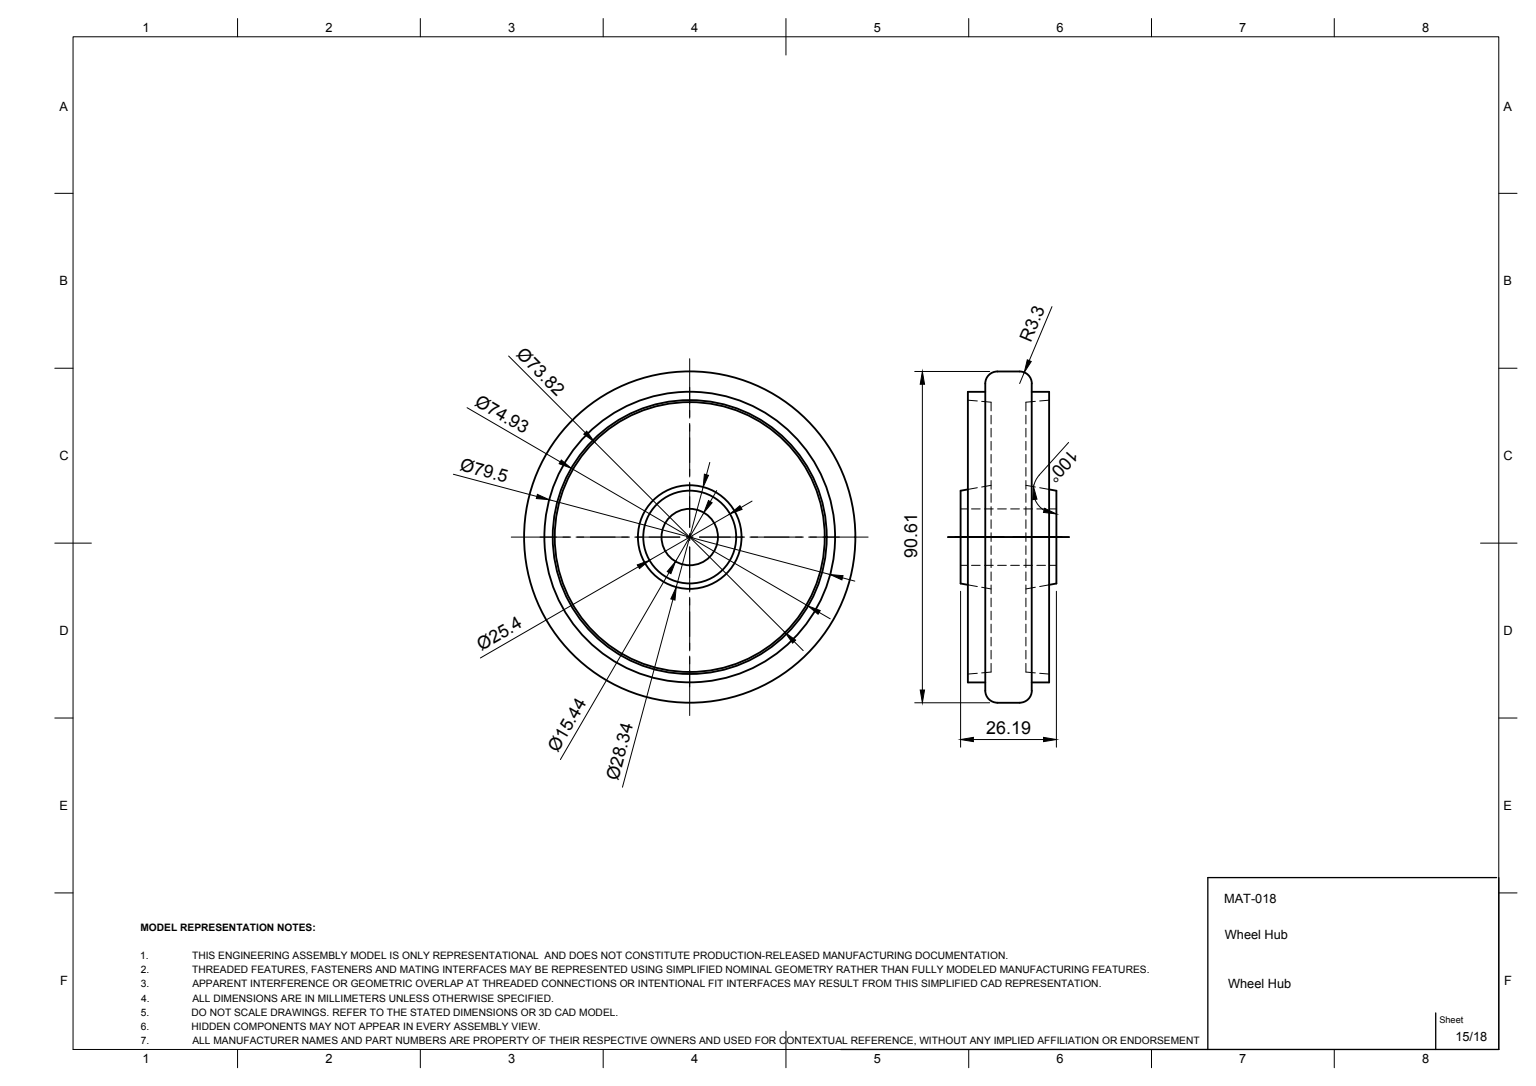
ISO-10303-21;
HEADER;
/* Generated by software containing ST-Developer
 * from STEP Tools, Inc. (www.steptools.com) 
 */

FILE_DESCRIPTION(
/* description */ ('STEP AP214'),
/* implementation_level */ '2;1');

FILE_NAME(
/* name */ 'Wheel Hub.step',
/* time_stamp */ '2026-11-14T06:16:09-08:00',
/* author */ (''),
/* organization */ (''),
/* preprocessor_version */ 'ST-DEVELOPER v20.2',
/* originating_system */ 'Autodesk Translation Framework v15.17.0.0',
/* authorisation */ '');

FILE_SCHEMA (('AUTOMOTIVE_DESIGN { 1 0 10303 214 3 1 1 }'));
ENDSEC;

DATA;
#10=MECHANICAL_DESIGN_GEOMETRIC_PRESENTATION_REPRESENTATION('',(#359),#18006);
#143=CONICAL_SURFACE('',#10734,12.7,0.174532925199433);
#144=CONICAL_SURFACE('',#10737,36.9094469866104,0.0872664625997163);
#145=CONICAL_SURFACE('',#10755,37.465,0.0872664625997151);
#146=CONICAL_SURFACE('',#10758,14.1695751798421,0.174532925199433);
#260=TOROIDAL_SURFACE('',#10743,42.00525,3.302);
#261=TOROIDAL_SURFACE('',#10749,42.00525,3.302);
#327=SHAPE_REPRESENTATION_RELATIONSHIP('SRR','None',#18085,#343);
#343=ADVANCED_BREP_SHAPE_REPRESENTATION('',(#375),#18002);
#359=STYLED_ITEM('',(#18170),#375);
#375=MANIFOLD_SOLID_BREP('Body1',#9568);
#486=FACE_BOUND('',#2066,.T.);
#487=FACE_BOUND('',#2068,.T.);
#488=FACE_BOUND('',#2070,.T.);
#489=FACE_BOUND('',#2072,.T.);
#490=FACE_BOUND('',#2074,.T.);
#491=FACE_BOUND('',#2076,.T.);
#492=FACE_BOUND('',#2078,.T.);
#493=FACE_BOUND('',#2080,.T.);
#825=PLANE('',#10764);
#826=PLANE('',#10765);
#827=PLANE('',#10766);
#828=PLANE('',#10767);
#829=PLANE('',#10768);
#830=PLANE('',#10769);
#831=PLANE('',#10770);
#832=PLANE('',#10771);
#1372=FACE_OUTER_BOUND('',#2055,.T.);
#1373=FACE_OUTER_BOUND('',#2056,.T.);
#1374=FACE_OUTER_BOUND('',#2057,.T.);
#1375=FACE_OUTER_BOUND('',#2058,.T.);
#1376=FACE_OUTER_BOUND('',#2059,.T.);
#1377=FACE_OUTER_BOUND('',#2060,.T.);
#1378=FACE_OUTER_BOUND('',#2061,.T.);
#1379=FACE_OUTER_BOUND('',#2062,.T.);
#1380=FACE_OUTER_BOUND('',#2063,.T.);
#1381=FACE_OUTER_BOUND('',#2064,.T.);
#1382=FACE_OUTER_BOUND('',#2065,.T.);
#1383=FACE_OUTER_BOUND('',#2067,.T.);
#1384=FACE_OUTER_BOUND('',#2069,.T.);
#1385=FACE_OUTER_BOUND('',#2071,.T.);
#1386=FACE_OUTER_BOUND('',#2073,.T.);
#1387=FACE_OUTER_BOUND('',#2075,.T.);
#1388=FACE_OUTER_BOUND('',#2077,.T.);
#1389=FACE_OUTER_BOUND('',#2079,.T.);
#2055=EDGE_LOOP('',(#8650,#8651,#8652,#8653));
#2056=EDGE_LOOP('',(#8654,#8655,#8656,#8657));
#2057=EDGE_LOOP('',(#8658,#8659,#8660,#8661));
#2058=EDGE_LOOP('',(#8662,#8663,#8664,#8665));
#2059=EDGE_LOOP('',(#8666,#8667,#8668,#8669));
#2060=EDGE_LOOP('',(#8670,#8671,#8672,#8673));
#2061=EDGE_LOOP('',(#8674,#8675,#8676,#8677));
#2062=EDGE_LOOP('',(#8678,#8679,#8680,#8681));
#2063=EDGE_LOOP('',(#8682,#8683,#8684,#8685));
#2064=EDGE_LOOP('',(#8686,#8687,#8688,#8689));
#2065=EDGE_LOOP('',(#8690));
#2066=EDGE_LOOP('',(#8691));
#2067=EDGE_LOOP('',(#8692));
#2068=EDGE_LOOP('',(#8693));
#2069=EDGE_LOOP('',(#8694));
#2070=EDGE_LOOP('',(#8695));
#2071=EDGE_LOOP('',(#8696));
#2072=EDGE_LOOP('',(#8697));
#2073=EDGE_LOOP('',(#8698));
#2074=EDGE_LOOP('',(#8699));
#2075=EDGE_LOOP('',(#8700));
#2076=EDGE_LOOP('',(#8701));
#2077=EDGE_LOOP('',(#8702));
#2078=EDGE_LOOP('',(#8703));
#2079=EDGE_LOOP('',(#8704));
#2080=EDGE_LOOP('',(#8705));
#2819=LINE('',#17773,#3543);
#2820=LINE('',#17779,#3544);
#2821=LINE('',#17785,#3545);
#2822=LINE('',#17796,#3546);
#2823=LINE('',#17805,#3547);
#2824=LINE('',#17811,#3548);
#2825=LINE('',#17817,#3549);
#2826=LINE('',#17823,#3550);
#3543=VECTOR('',#13538,12.7);
#3544=VECTOR('',#13545,36.9094469866104);
#3545=VECTOR('',#13552,39.751);
#3546=VECTOR('',#13567,45.30725);
#3547=VECTOR('',#13578,39.751);
#3548=VECTOR('',#13585,37.465);
#3549=VECTOR('',#13592,14.1695751798421);
#3550=VECTOR('',#13599,7.7216);
#3955=CIRCLE('',#10735,14.1695751798421);
#3956=CIRCLE('',#10736,12.7);
#3957=CIRCLE('',#10738,36.9094469866104);
#3958=CIRCLE('',#10739,37.465);
#3959=CIRCLE('',#10741,39.751);
#3960=CIRCLE('',#10742,39.751);
#3961=CIRCLE('',#10744,45.30725);
#3962=CIRCLE('',#10745,3.302);
#3963=CIRCLE('',#10746,42.00525);
#3964=CIRCLE('',#10748,45.30725);
#3965=CIRCLE('',#10750,42.00525);
#3966=CIRCLE('',#10751,3.302);
#3967=CIRCLE('',#10753,39.751);
#3968=CIRCLE('',#10754,39.751);
#3969=CIRCLE('',#10756,36.9094469866104);
#3970=CIRCLE('',#10757,37.465);
#3971=CIRCLE('',#10759,14.1695751798421);
#3972=CIRCLE('',#10760,12.7);
#3973=CIRCLE('',#10762,7.7216);
#3974=CIRCLE('',#10763,7.7216);
#4774=VERTEX_POINT('',#17770);
#4775=VERTEX_POINT('',#17772);
#4776=VERTEX_POINT('',#17776);
#4777=VERTEX_POINT('',#17778);
#4778=VERTEX_POINT('',#17782);
#4779=VERTEX_POINT('',#17784);
#4780=VERTEX_POINT('',#17788);
#4781=VERTEX_POINT('',#17790);
#4782=VERTEX_POINT('',#17794);
#4783=VERTEX_POINT('',#17798);
#4784=VERTEX_POINT('',#17802);
#4785=VERTEX_POINT('',#17804);
#4786=VERTEX_POINT('',#17808);
#4787=VERTEX_POINT('',#17810);
#4788=VERTEX_POINT('',#17814);
#4789=VERTEX_POINT('',#17816);
#4790=VERTEX_POINT('',#17820);
#4791=VERTEX_POINT('',#17822);
#6073=EDGE_CURVE('',#4774,#4774,#3955,.T.);
#6074=EDGE_CURVE('',#4774,#4775,#2819,.T.);
#6075=EDGE_CURVE('',#4775,#4775,#3956,.T.);
#6076=EDGE_CURVE('',#4776,#4776,#3957,.T.);
#6077=EDGE_CURVE('',#4776,#4777,#2820,.T.);
#6078=EDGE_CURVE('',#4777,#4777,#3958,.T.);
#6079=EDGE_CURVE('',#4778,#4778,#3959,.T.);
#6080=EDGE_CURVE('',#4778,#4779,#2821,.T.);
#6081=EDGE_CURVE('',#4779,#4779,#3960,.T.);
#6082=EDGE_CURVE('',#4780,#4780,#3961,.T.);
#6083=EDGE_CURVE('',#4780,#4781,#3962,.T.);
#6084=EDGE_CURVE('',#4781,#4781,#3963,.T.);
#6085=EDGE_CURVE('',#4782,#4782,#3964,.T.);
#6086=EDGE_CURVE('',#4782,#4780,#2822,.T.);
#6087=EDGE_CURVE('',#4783,#4783,#3965,.T.);
#6088=EDGE_CURVE('',#4783,#4782,#3966,.T.);
#6089=EDGE_CURVE('',#4784,#4784,#3967,.T.);
#6090=EDGE_CURVE('',#4784,#4785,#2823,.T.);
#6091=EDGE_CURVE('',#4785,#4785,#3968,.T.);
#6092=EDGE_CURVE('',#4786,#4786,#3969,.T.);
#6093=EDGE_CURVE('',#4786,#4787,#2824,.T.);
#6094=EDGE_CURVE('',#4787,#4787,#3970,.T.);
#6095=EDGE_CURVE('',#4788,#4788,#3971,.T.);
#6096=EDGE_CURVE('',#4788,#4789,#2825,.T.);
#6097=EDGE_CURVE('',#4789,#4789,#3972,.T.);
#6098=EDGE_CURVE('',#4790,#4790,#3973,.T.);
#6099=EDGE_CURVE('',#4790,#4791,#2826,.T.);
#6100=EDGE_CURVE('',#4791,#4791,#3974,.T.);
#8650=ORIENTED_EDGE('',*,*,#6073,.F.);
#8651=ORIENTED_EDGE('',*,*,#6074,.T.);
#8652=ORIENTED_EDGE('',*,*,#6075,.T.);
#8653=ORIENTED_EDGE('',*,*,#6074,.F.);
#8654=ORIENTED_EDGE('',*,*,#6076,.T.);
#8655=ORIENTED_EDGE('',*,*,#6077,.T.);
#8656=ORIENTED_EDGE('',*,*,#6078,.F.);
#8657=ORIENTED_EDGE('',*,*,#6077,.F.);
#8658=ORIENTED_EDGE('',*,*,#6079,.F.);
#8659=ORIENTED_EDGE('',*,*,#6080,.T.);
#8660=ORIENTED_EDGE('',*,*,#6081,.T.);
#8661=ORIENTED_EDGE('',*,*,#6080,.F.);
#8662=ORIENTED_EDGE('',*,*,#6082,.F.);
#8663=ORIENTED_EDGE('',*,*,#6083,.T.);
#8664=ORIENTED_EDGE('',*,*,#6084,.T.);
#8665=ORIENTED_EDGE('',*,*,#6083,.F.);
#8666=ORIENTED_EDGE('',*,*,#6085,.F.);
#8667=ORIENTED_EDGE('',*,*,#6086,.T.);
#8668=ORIENTED_EDGE('',*,*,#6082,.T.);
#8669=ORIENTED_EDGE('',*,*,#6086,.F.);
#8670=ORIENTED_EDGE('',*,*,#6087,.F.);
#8671=ORIENTED_EDGE('',*,*,#6088,.T.);
#8672=ORIENTED_EDGE('',*,*,#6085,.T.);
#8673=ORIENTED_EDGE('',*,*,#6088,.F.);
#8674=ORIENTED_EDGE('',*,*,#6089,.F.);
#8675=ORIENTED_EDGE('',*,*,#6090,.T.);
#8676=ORIENTED_EDGE('',*,*,#6091,.T.);
#8677=ORIENTED_EDGE('',*,*,#6090,.F.);
#8678=ORIENTED_EDGE('',*,*,#6092,.F.);
#8679=ORIENTED_EDGE('',*,*,#6093,.T.);
#8680=ORIENTED_EDGE('',*,*,#6094,.T.);
#8681=ORIENTED_EDGE('',*,*,#6093,.F.);
#8682=ORIENTED_EDGE('',*,*,#6095,.T.);
#8683=ORIENTED_EDGE('',*,*,#6096,.T.);
#8684=ORIENTED_EDGE('',*,*,#6097,.F.);
#8685=ORIENTED_EDGE('',*,*,#6096,.F.);
#8686=ORIENTED_EDGE('',*,*,#6098,.F.);
#8687=ORIENTED_EDGE('',*,*,#6099,.T.);
#8688=ORIENTED_EDGE('',*,*,#6100,.T.);
#8689=ORIENTED_EDGE('',*,*,#6099,.F.);
#8690=ORIENTED_EDGE('',*,*,#6097,.T.);
#8691=ORIENTED_EDGE('',*,*,#6100,.F.);
#8692=ORIENTED_EDGE('',*,*,#6092,.T.);
#8693=ORIENTED_EDGE('',*,*,#6095,.F.);
#8694=ORIENTED_EDGE('',*,*,#6089,.T.);
#8695=ORIENTED_EDGE('',*,*,#6094,.F.);
#8696=ORIENTED_EDGE('',*,*,#6087,.T.);
#8697=ORIENTED_EDGE('',*,*,#6091,.F.);
#8698=ORIENTED_EDGE('',*,*,#6084,.F.);
#8699=ORIENTED_EDGE('',*,*,#6079,.T.);
#8700=ORIENTED_EDGE('',*,*,#6081,.F.);
#8701=ORIENTED_EDGE('',*,*,#6078,.T.);
#8702=ORIENTED_EDGE('',*,*,#6076,.F.);
#8703=ORIENTED_EDGE('',*,*,#6073,.T.);
#8704=ORIENTED_EDGE('',*,*,#6075,.F.);
#8705=ORIENTED_EDGE('',*,*,#6098,.T.);
#8969=CYLINDRICAL_SURFACE('',#10740,39.751);
#8970=CYLINDRICAL_SURFACE('',#10747,45.30725);
#8971=CYLINDRICAL_SURFACE('',#10752,39.751);
#8972=CYLINDRICAL_SURFACE('',#10761,7.7216);
#9511=ADVANCED_FACE('',(#1372),#143,.T.);
#9512=ADVANCED_FACE('',(#1373),#144,.F.);
#9513=ADVANCED_FACE('',(#1374),#8969,.T.);
#9514=ADVANCED_FACE('',(#1375),#260,.T.);
#9515=ADVANCED_FACE('',(#1376),#8970,.T.);
#9516=ADVANCED_FACE('',(#1377),#261,.T.);
#9517=ADVANCED_FACE('',(#1378),#8971,.T.);
#9518=ADVANCED_FACE('',(#1379),#145,.F.);
#9519=ADVANCED_FACE('',(#1380),#146,.T.);
#9520=ADVANCED_FACE('',(#1381),#8972,.F.);
#9521=ADVANCED_FACE('',(#1382,#486),#825,.F.);
#9522=ADVANCED_FACE('',(#1383,#487),#826,.F.);
#9523=ADVANCED_FACE('',(#1384,#488),#827,.F.);
#9524=ADVANCED_FACE('',(#1385,#489),#828,.F.);
#9525=ADVANCED_FACE('',(#1386,#490),#829,.F.);
#9526=ADVANCED_FACE('',(#1387,#491),#830,.F.);
#9527=ADVANCED_FACE('',(#1388,#492),#831,.F.);
#9528=ADVANCED_FACE('',(#1389,#493),#832,.F.);
#9568=CLOSED_SHELL('',(#9511,#9512,#9513,#9514,#9515,#9516,#9517,#9518,
#9519,#9520,#9521,#9522,#9523,#9524,#9525,#9526,#9527,#9528));
#10733=AXIS2_PLACEMENT_3D('',#17768,#13532,#13533);
#10734=AXIS2_PLACEMENT_3D('',#17769,#13534,#13535);
#10735=AXIS2_PLACEMENT_3D('',#17771,#13536,#13537);
#10736=AXIS2_PLACEMENT_3D('',#17774,#13539,#13540);
#10737=AXIS2_PLACEMENT_3D('',#17775,#13541,#13542);
#10738=AXIS2_PLACEMENT_3D('',#17777,#13543,#13544);
#10739=AXIS2_PLACEMENT_3D('',#17780,#13546,#13547);
#10740=AXIS2_PLACEMENT_3D('',#17781,#13548,#13549);
#10741=AXIS2_PLACEMENT_3D('',#17783,#13550,#13551);
#10742=AXIS2_PLACEMENT_3D('',#17786,#13553,#13554);
#10743=AXIS2_PLACEMENT_3D('',#17787,#13555,#13556);
#10744=AXIS2_PLACEMENT_3D('',#17789,#13557,#13558);
#10745=AXIS2_PLACEMENT_3D('',#17791,#13559,#13560);
#10746=AXIS2_PLACEMENT_3D('',#17792,#13561,#13562);
#10747=AXIS2_PLACEMENT_3D('',#17793,#13563,#13564);
#10748=AXIS2_PLACEMENT_3D('',#17795,#13565,#13566);
#10749=AXIS2_PLACEMENT_3D('',#17797,#13568,#13569);
#10750=AXIS2_PLACEMENT_3D('',#17799,#13570,#13571);
#10751=AXIS2_PLACEMENT_3D('',#17800,#13572,#13573);
#10752=AXIS2_PLACEMENT_3D('',#17801,#13574,#13575);
#10753=AXIS2_PLACEMENT_3D('',#17803,#13576,#13577);
#10754=AXIS2_PLACEMENT_3D('',#17806,#13579,#13580);
#10755=AXIS2_PLACEMENT_3D('',#17807,#13581,#13582);
#10756=AXIS2_PLACEMENT_3D('',#17809,#13583,#13584);
#10757=AXIS2_PLACEMENT_3D('',#17812,#13586,#13587);
#10758=AXIS2_PLACEMENT_3D('',#17813,#13588,#13589);
#10759=AXIS2_PLACEMENT_3D('',#17815,#13590,#13591);
#10760=AXIS2_PLACEMENT_3D('',#17818,#13593,#13594);
#10761=AXIS2_PLACEMENT_3D('',#17819,#13595,#13596);
#10762=AXIS2_PLACEMENT_3D('',#17821,#13597,#13598);
#10763=AXIS2_PLACEMENT_3D('',#17824,#13600,#13601);
#10764=AXIS2_PLACEMENT_3D('',#17825,#13602,#13603);
#10765=AXIS2_PLACEMENT_3D('',#17826,#13604,#13605);
#10766=AXIS2_PLACEMENT_3D('',#17827,#13606,#13607);
#10767=AXIS2_PLACEMENT_3D('',#17828,#13608,#13609);
#10768=AXIS2_PLACEMENT_3D('',#17829,#13610,#13611);
#10769=AXIS2_PLACEMENT_3D('',#17830,#13612,#13613);
#10770=AXIS2_PLACEMENT_3D('',#17831,#13614,#13615);
#10771=AXIS2_PLACEMENT_3D('',#17832,#13616,#13617);
#13532=DIRECTION('axis',(0.,0.,1.));
#13533=DIRECTION('refdir',(1.,0.,0.));
#13534=DIRECTION('center_axis',(0.,0.,-1.));
#13535=DIRECTION('ref_axis',(-1.,0.,0.));
#13536=DIRECTION('center_axis',(0.,0.,-1.));
#13537=DIRECTION('ref_axis',(-1.,0.,0.));
#13538=DIRECTION('',(-0.173648177666931,2.12657684957577E-17,0.984807753012208));
#13539=DIRECTION('center_axis',(0.,0.,-1.));
#13540=DIRECTION('ref_axis',(-1.,0.,0.));
#13541=DIRECTION('center_axis',(0.,0.,1.));
#13542=DIRECTION('ref_axis',(1.,0.,0.));
#13543=DIRECTION('center_axis',(0.,0.,-1.));
#13544=DIRECTION('ref_axis',(-1.,0.,0.));
#13545=DIRECTION('',(-0.087155742747658,-1.06735001383229E-17,0.996194698091746));
#13546=DIRECTION('center_axis',(0.,0.,-1.));
#13547=DIRECTION('ref_axis',(-1.,0.,0.));
#13548=DIRECTION('center_axis',(0.,0.,-1.));
#13549=DIRECTION('ref_axis',(-1.,0.,0.));
#13550=DIRECTION('center_axis',(0.,0.,-1.));
#13551=DIRECTION('ref_axis',(-1.,0.,0.));
#13552=DIRECTION('',(0.,0.,1.));
#13553=DIRECTION('center_axis',(0.,0.,-1.));
#13554=DIRECTION('ref_axis',(-1.,0.,0.));
#13555=DIRECTION('center_axis',(0.,0.,-1.));
#13556=DIRECTION('ref_axis',(-1.,0.,0.));
#13557=DIRECTION('center_axis',(0.,0.,-1.));
#13558=DIRECTION('ref_axis',(-1.,0.,0.));
#13559=DIRECTION('center_axis',(-1.22464679914735E-16,-1.,0.));
#13560=DIRECTION('ref_axis',(1.,-1.22464679914735E-16,0.));
#13561=DIRECTION('center_axis',(0.,0.,-1.));
#13562=DIRECTION('ref_axis',(-1.,0.,0.));
#13563=DIRECTION('center_axis',(0.,0.,-1.));
#13564=DIRECTION('ref_axis',(-1.,0.,0.));
#13565=DIRECTION('center_axis',(0.,0.,-1.));
#13566=DIRECTION('ref_axis',(-1.,0.,0.));
#13567=DIRECTION('',(0.,0.,1.));
#13568=DIRECTION('center_axis',(0.,0.,-1.));
#13569=DIRECTION('ref_axis',(-1.,0.,0.));
#13570=DIRECTION('center_axis',(0.,0.,-1.));
#13571=DIRECTION('ref_axis',(-1.,0.,0.));
#13572=DIRECTION('center_axis',(-1.22464679914735E-16,-1.,0.));
#13573=DIRECTION('ref_axis',(1.,-1.22464679914735E-16,0.));
#13574=DIRECTION('center_axis',(0.,0.,-1.));
#13575=DIRECTION('ref_axis',(-1.,0.,0.));
#13576=DIRECTION('center_axis',(0.,0.,-1.));
#13577=DIRECTION('ref_axis',(-1.,0.,0.));
#13578=DIRECTION('',(0.,0.,1.));
#13579=DIRECTION('center_axis',(0.,0.,-1.));
#13580=DIRECTION('ref_axis',(-1.,0.,0.));
#13581=DIRECTION('center_axis',(0.,0.,-1.));
#13582=DIRECTION('ref_axis',(-1.,0.,0.));
#13583=DIRECTION('center_axis',(0.,0.,-1.));
#13584=DIRECTION('ref_axis',(-1.,0.,0.));
#13585=DIRECTION('',(0.0871557427476568,-1.06735001383228E-17,-0.996194698091746));
#13586=DIRECTION('center_axis',(0.,0.,-1.));
#13587=DIRECTION('ref_axis',(-1.,0.,0.));
#13588=DIRECTION('center_axis',(0.,0.,1.));
#13589=DIRECTION('ref_axis',(1.,0.,0.));
#13590=DIRECTION('center_axis',(0.,0.,-1.));
#13591=DIRECTION('ref_axis',(-1.,0.,0.));
#13592=DIRECTION('',(0.173648177666931,2.12657684957577E-17,-0.984807753012208));
#13593=DIRECTION('center_axis',(0.,0.,-1.));
#13594=DIRECTION('ref_axis',(-1.,0.,0.));
#13595=DIRECTION('center_axis',(0.,0.,-1.));
#13596=DIRECTION('ref_axis',(-1.,0.,0.));
#13597=DIRECTION('center_axis',(0.,0.,-1.));
#13598=DIRECTION('ref_axis',(-1.,0.,0.));
#13599=DIRECTION('',(0.,0.,-1.));
#13600=DIRECTION('center_axis',(0.,0.,-1.));
#13601=DIRECTION('ref_axis',(-1.,0.,0.));
#13602=DIRECTION('center_axis',(0.,0.,1.));
#13603=DIRECTION('ref_axis',(1.,0.,0.));
#13604=DIRECTION('center_axis',(0.,0.,1.));
#13605=DIRECTION('ref_axis',(1.,0.,0.));
#13606=DIRECTION('center_axis',(0.,0.,1.));
#13607=DIRECTION('ref_axis',(1.,0.,0.));
#13608=DIRECTION('center_axis',(0.,0.,1.));
#13609=DIRECTION('ref_axis',(1.,0.,0.));
#13610=DIRECTION('center_axis',(0.,0.,-1.));
#13611=DIRECTION('ref_axis',(0.,-1.,0.));
#13612=DIRECTION('center_axis',(0.,0.,-1.));
#13613=DIRECTION('ref_axis',(0.,-1.,0.));
#13614=DIRECTION('center_axis',(0.,0.,-1.));
#13615=DIRECTION('ref_axis',(0.,-1.,0.));
#13616=DIRECTION('center_axis',(0.,0.,-1.));
#13617=DIRECTION('ref_axis',(0.,-1.,0.));
#17768=CARTESIAN_POINT('',(0.,0.,0.));
#17769=CARTESIAN_POINT('Origin',(0.,0.,13.096875));
#17770=CARTESIAN_POINT('',(14.1695751798421,-1.73527248892714E-15,4.7625));
#17771=CARTESIAN_POINT('Origin',(6.93889390390723E-15,0.,4.7625));
#17772=CARTESIAN_POINT('',(12.7,-1.55530143491714E-15,13.096875));
#17773=CARTESIAN_POINT('',(12.7,-1.55530143491714E-15,13.096875));
#17774=CARTESIAN_POINT('Origin',(0.,0.,13.096875));
#17775=CARTESIAN_POINT('Origin',(6.93889390390723E-15,0.,4.7625));
#17776=CARTESIAN_POINT('',(-36.9094469866104,-4.52010361104513E-15,4.7625));
#17777=CARTESIAN_POINT('Origin',(6.93889390390723E-15,0.,4.7625));
#17778=CARTESIAN_POINT('',(-37.465,-4.58813923300556E-15,11.1125));
#17779=CARTESIAN_POINT('',(-36.9094469866104,-4.52010361104513E-15,4.7625));
#17780=CARTESIAN_POINT('Origin',(0.,0.,11.1125));
#17781=CARTESIAN_POINT('Origin',(-1.10328413072125E-12,0.,-13.096875));
#17782=CARTESIAN_POINT('',(39.7509999999989,-4.86809349129064E-15,6.35000000000002));
#17783=CARTESIAN_POINT('Origin',(-1.11022302462516E-12,0.,6.35000000000002));
#17784=CARTESIAN_POINT('',(39.7509999999989,-4.86809349129064E-15,11.1125));
#17785=CARTESIAN_POINT('',(39.7509999999989,-4.86809349129064E-15,-13.096875));
#17786=CARTESIAN_POINT('Origin',(0.,0.,11.1125));
#17787=CARTESIAN_POINT('Origin',(0.,0.,3.048));
#17788=CARTESIAN_POINT('',(45.30725,-5.54853786906689E-15,3.048));
#17789=CARTESIAN_POINT('Origin',(0.,0.,3.048));
#17790=CARTESIAN_POINT('',(42.0052499999989,-5.1441594959883E-15,6.35000000000002));
#17791=CARTESIAN_POINT('Origin',(42.00525,-5.14415949598844E-15,3.048));
#17792=CARTESIAN_POINT('Origin',(-1.11022302462516E-12,0.,6.35000000000002));
#17793=CARTESIAN_POINT('Origin',(-1.10328413072125E-12,0.,-13.096875));
#17794=CARTESIAN_POINT('',(45.3072499999989,-5.54853786906689E-15,-3.048));
#17795=CARTESIAN_POINT('Origin',(-1.10328413072125E-12,0.,-3.048));
#17796=CARTESIAN_POINT('',(45.3072499999989,-5.54853786906689E-15,-13.096875));
#17797=CARTESIAN_POINT('Origin',(-1.10328413072125E-12,0.,-3.048));
#17798=CARTESIAN_POINT('',(42.00525,-5.14415949598857E-15,-6.35000000000002));
#17799=CARTESIAN_POINT('Origin',(6.93889390390723E-15,0.,-6.35000000000002));
#17800=CARTESIAN_POINT('Origin',(42.0052499999989,-5.14415949598844E-15,
-3.048));
#17801=CARTESIAN_POINT('Origin',(-1.10328413072125E-12,0.,-13.096875));
#17802=CARTESIAN_POINT('',(39.7509999999989,-4.86809349129064E-15,-11.1125));
#17803=CARTESIAN_POINT('Origin',(-1.10328413072125E-12,0.,-11.1125));
#17804=CARTESIAN_POINT('',(39.7509999999989,-4.86809349129064E-15,-6.35000000000002));
#17805=CARTESIAN_POINT('',(39.7509999999989,-4.86809349129064E-15,-13.096875));
#17806=CARTESIAN_POINT('Origin',(6.93889390390723E-15,0.,-6.35000000000002));
#17807=CARTESIAN_POINT('Origin',(-1.10328413072125E-12,0.,-11.1125));
#17808=CARTESIAN_POINT('',(36.9094469866093,-4.52010361104513E-15,-4.7625));
#17809=CARTESIAN_POINT('Origin',(-1.11022302462516E-12,0.,-4.7625));
#17810=CARTESIAN_POINT('',(37.4649999999989,-4.58813923300556E-15,-11.1125));
#17811=CARTESIAN_POINT('',(37.4649999999989,-4.58813923300556E-15,-11.1125));
#17812=CARTESIAN_POINT('Origin',(-1.10328413072125E-12,0.,-11.1125));
#17813=CARTESIAN_POINT('Origin',(-1.11022302462516E-12,0.,-4.7625));
#17814=CARTESIAN_POINT('',(-14.1695751798432,-1.73527248892714E-15,-4.7625));
#17815=CARTESIAN_POINT('Origin',(-1.11022302462516E-12,0.,-4.7625));
#17816=CARTESIAN_POINT('',(-12.7000000000011,-1.55530143491714E-15,-13.096875));
#17817=CARTESIAN_POINT('',(-14.1695751798432,-1.73527248892714E-15,-4.7625));
#17818=CARTESIAN_POINT('Origin',(-1.10328413072125E-12,0.,-13.096875));
#17819=CARTESIAN_POINT('Origin',(-1.10328413072125E-12,0.,-13.096875));
#17820=CARTESIAN_POINT('',(7.7215999999989,-9.4562327242962E-16,13.096875));
#17821=CARTESIAN_POINT('Origin',(0.,0.,13.096875));
#17822=CARTESIAN_POINT('',(7.7215999999989,-9.4562327242962E-16,-13.096875));
#17823=CARTESIAN_POINT('',(7.7215999999989,-9.4562327242962E-16,-13.096875));
#17824=CARTESIAN_POINT('Origin',(-1.10328413072125E-12,0.,-13.096875));
#17825=CARTESIAN_POINT('Origin',(-1.10328413072125E-12,12.7,-13.096875));
#17826=CARTESIAN_POINT('Origin',(-1.11022302462516E-12,36.9094469866104,
-4.7625));
#17827=CARTESIAN_POINT('Origin',(-1.10328413072125E-12,39.751,-11.1125));
#17828=CARTESIAN_POINT('Origin',(6.93889390390723E-15,42.00525,-6.35000000000002));
#17829=CARTESIAN_POINT('Origin',(-1.11022302462516E-12,39.751,6.35000000000002));
#17830=CARTESIAN_POINT('Origin',(0.,37.465,11.1125));
#17831=CARTESIAN_POINT('Origin',(6.93889390390723E-15,14.1695751798421,
4.7625));
#17832=CARTESIAN_POINT('Origin',(0.,0.,13.096875));
#17982=UNCERTAINTY_MEASURE_WITH_UNIT(LENGTH_MEASURE(0.01),#18007,
'DISTANCE_ACCURACY_VALUE',
'Maximum model space distance between geometric entities at asserted c
onnectivities');
#17986=UNCERTAINTY_MEASURE_WITH_UNIT(LENGTH_MEASURE(0.01),#18007,
'DISTANCE_ACCURACY_VALUE',
'Maximum model space distance between geometric entities at asserted c
onnectivities');
#18002=(
GEOMETRIC_REPRESENTATION_CONTEXT(3)
GLOBAL_UNCERTAINTY_ASSIGNED_CONTEXT((#17982))
GLOBAL_UNIT_ASSIGNED_CONTEXT((#18007,#18009,#18010))
REPRESENTATION_CONTEXT('','3D')
);
#18006=(
GEOMETRIC_REPRESENTATION_CONTEXT(3)
GLOBAL_UNCERTAINTY_ASSIGNED_CONTEXT((#17986))
GLOBAL_UNIT_ASSIGNED_CONTEXT((#18007,#18009,#18010))
REPRESENTATION_CONTEXT('','3D')
);
#18007=(
LENGTH_UNIT()
NAMED_UNIT(*)
SI_UNIT(.MILLI.,.METRE.)
);
#18009=(
NAMED_UNIT(*)
PLANE_ANGLE_UNIT()
SI_UNIT($,.RADIAN.)
);
#18010=(
NAMED_UNIT(*)
SI_UNIT($,.STERADIAN.)
SOLID_ANGLE_UNIT()
);
#18026=SHAPE_DEFINITION_REPRESENTATION(#18045,#18085);
#18045=PRODUCT_DEFINITION_SHAPE('',$,#18105);
#18085=SHAPE_REPRESENTATION('',(#10733),#18002);
#18089=PRODUCT_DEFINITION_CONTEXT('part definition',#18148,'design');
#18105=PRODUCT_DEFINITION('Wheel Hub','Wheel Hub',#18124,#18089);
#18124=PRODUCT_DEFINITION_FORMATION('',$,#18165);
#18148=APPLICATION_CONTEXT(
'Core Data for Automotive Mechanical Design Process');
#18149=PRODUCT_CONTEXT('part definition',#18148,'mechanical');
#18165=PRODUCT('Wheel Hub','Wheel Hub',$,(#18149));
#18170=PRESENTATION_STYLE_ASSIGNMENT((#18174));
#18174=SURFACE_STYLE_USAGE(.BOTH.,#18178);
#18178=SURFACE_SIDE_STYLE('',(#18182));
#18182=SURFACE_STYLE_FILL_AREA(#18186);
#18186=FILL_AREA_STYLE('Opaque(227,224,212)',(#18190));
#18190=FILL_AREA_STYLE_COLOUR('Opaque(227,224,212)',#18194);
#18194=COLOUR_RGB('Opaque(227,224,212)',0.890196078431372,0.87843137254902,
0.831372549019608);
ENDSEC;
END-ISO-10303-21;
